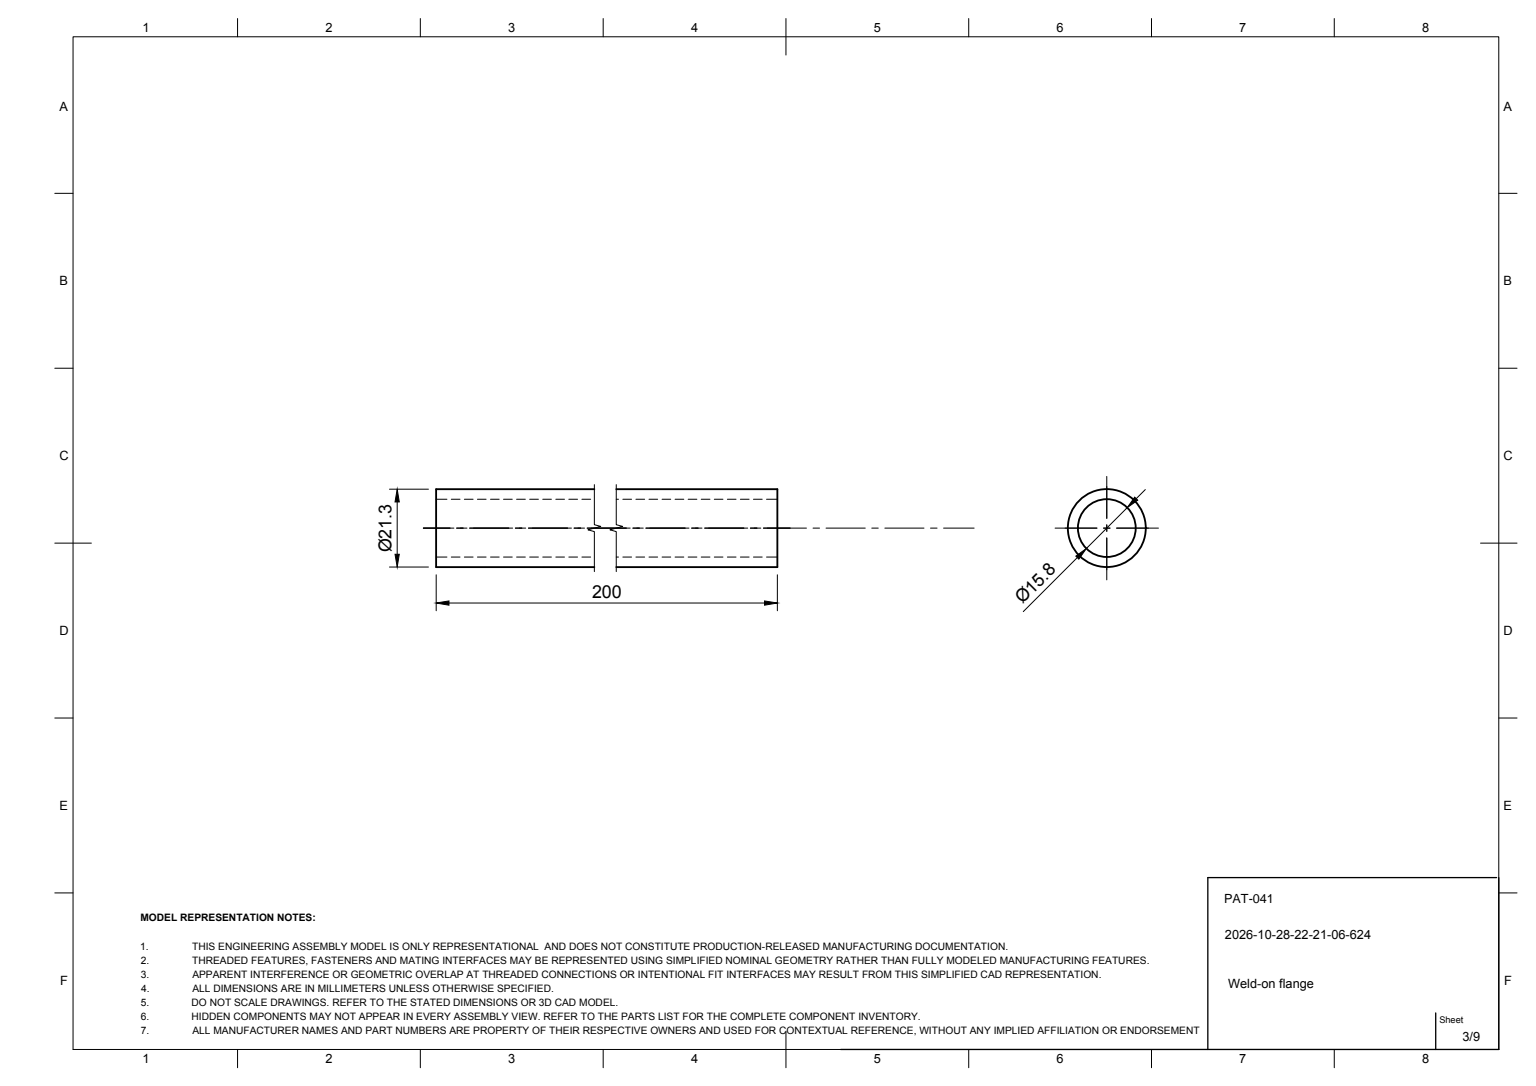
ISO-10303-21;
HEADER;
/* Generated by software containing ST-Developer
 * from STEP Tools, Inc. (www.steptools.com) 
 */

FILE_DESCRIPTION(
/* description */ ('PAT-041'),
/* implementation_level */ '2;1');

FILE_NAME(
/* name */ 'Weld-on flange.step',
/* time_stamp */ '2026-10-28T22:21:24-07:00',
/* author */ (''),
/* organization */ (''),
/* preprocessor_version */ 'ST-DEVELOPER v20.2',
/* originating_system */ 'Autodesk Translation Framework v15.17.0.0',
/* authorisation */ '');

FILE_SCHEMA (('AUTOMOTIVE_DESIGN { 1 0 10303 214 3 1 1 }'));
ENDSEC;

DATA;
#10=MECHANICAL_DESIGN_GEOMETRIC_PRESENTATION_REPRESENTATION('',(#210),#2507);
#190=SHAPE_REPRESENTATION_RELATIONSHIP('SRR','None',#2575,#200);
#200=ADVANCED_BREP_SHAPE_REPRESENTATION('',(#220),#2498);
#210=STYLED_ITEM('',(#2687),#220);
#220=MANIFOLD_SOLID_BREP('Body1',#1330);
#231=FACE_BOUND('',#397,.T.);
#232=FACE_BOUND('',#398,.T.);
#233=FACE_BOUND('',#399,.T.);
#234=FACE_BOUND('',#400,.T.);
#235=FACE_BOUND('',#401,.T.);
#236=FACE_BOUND('',#403,.T.);
#237=FACE_BOUND('',#404,.T.);
#238=FACE_BOUND('',#405,.T.);
#239=FACE_BOUND('',#406,.T.);
#240=FACE_BOUND('',#407,.T.);
#282=PLANE('',#1479);
#283=PLANE('',#1480);
#317=FACE_OUTER_BOUND('',#390,.T.);
#318=FACE_OUTER_BOUND('',#391,.T.);
#319=FACE_OUTER_BOUND('',#392,.T.);
#320=FACE_OUTER_BOUND('',#393,.T.);
#321=FACE_OUTER_BOUND('',#394,.T.);
#322=FACE_OUTER_BOUND('',#395,.T.);
#323=FACE_OUTER_BOUND('',#396,.T.);
#324=FACE_OUTER_BOUND('',#402,.T.);
#390=EDGE_LOOP('',(#944,#945,#946,#947));
#391=EDGE_LOOP('',(#948,#949,#950,#951));
#392=EDGE_LOOP('',(#952,#953,#954,#955));
#393=EDGE_LOOP('',(#956,#957,#958,#959));
#394=EDGE_LOOP('',(#960,#961,#962,#963));
#395=EDGE_LOOP('',(#964,#965,#966,#967));
#396=EDGE_LOOP('',(#968));
#397=EDGE_LOOP('',(#969));
#398=EDGE_LOOP('',(#970));
#399=EDGE_LOOP('',(#971));
#400=EDGE_LOOP('',(#972));
#401=EDGE_LOOP('',(#973));
#402=EDGE_LOOP('',(#974));
#403=EDGE_LOOP('',(#975));
#404=EDGE_LOOP('',(#976));
#405=EDGE_LOOP('',(#977));
#406=EDGE_LOOP('',(#978));
#407=EDGE_LOOP('',(#979));
#508=LINE('',#2106,#564);
#509=LINE('',#2112,#565);
#510=LINE('',#2118,#566);
#511=LINE('',#2124,#567);
#512=LINE('',#2130,#568);
#513=LINE('',#2136,#569);
#564=VECTOR('',#1671,0.44);
#565=VECTOR('',#1678,0.44);
#566=VECTOR('',#1685,0.44);
#567=VECTOR('',#1692,0.44);
#568=VECTOR('',#1699,1.065);
#569=VECTOR('',#1706,3.5);
#622=CIRCLE('',#1462,0.44);
#623=CIRCLE('',#1463,0.44);
#624=CIRCLE('',#1465,0.44);
#625=CIRCLE('',#1466,0.44);
#626=CIRCLE('',#1468,0.44);
#627=CIRCLE('',#1469,0.44);
#628=CIRCLE('',#1471,0.44);
#629=CIRCLE('',#1472,0.44);
#630=CIRCLE('',#1474,1.065);
#631=CIRCLE('',#1475,1.065);
#632=CIRCLE('',#1477,3.5);
#633=CIRCLE('',#1478,3.5);
#694=VERTEX_POINT('',#2103);
#695=VERTEX_POINT('',#2105);
#696=VERTEX_POINT('',#2109);
#697=VERTEX_POINT('',#2111);
#698=VERTEX_POINT('',#2115);
#699=VERTEX_POINT('',#2117);
#700=VERTEX_POINT('',#2121);
#701=VERTEX_POINT('',#2123);
#702=VERTEX_POINT('',#2127);
#703=VERTEX_POINT('',#2129);
#704=VERTEX_POINT('',#2133);
#705=VERTEX_POINT('',#2135);
#792=EDGE_CURVE('',#694,#694,#622,.T.);
#793=EDGE_CURVE('',#694,#695,#508,.T.);
#794=EDGE_CURVE('',#695,#695,#623,.T.);
#795=EDGE_CURVE('',#696,#696,#624,.T.);
#796=EDGE_CURVE('',#696,#697,#509,.T.);
#797=EDGE_CURVE('',#697,#697,#625,.T.);
#798=EDGE_CURVE('',#698,#698,#626,.T.);
#799=EDGE_CURVE('',#698,#699,#510,.T.);
#800=EDGE_CURVE('',#699,#699,#627,.T.);
#801=EDGE_CURVE('',#700,#700,#628,.T.);
#802=EDGE_CURVE('',#700,#701,#511,.T.);
#803=EDGE_CURVE('',#701,#701,#629,.T.);
#804=EDGE_CURVE('',#702,#702,#630,.T.);
#805=EDGE_CURVE('',#702,#703,#512,.T.);
#806=EDGE_CURVE('',#703,#703,#631,.T.);
#807=EDGE_CURVE('',#704,#704,#632,.T.);
#808=EDGE_CURVE('',#704,#705,#513,.T.);
#809=EDGE_CURVE('',#705,#705,#633,.T.);
#944=ORIENTED_EDGE('',*,*,#792,.F.);
#945=ORIENTED_EDGE('',*,*,#793,.T.);
#946=ORIENTED_EDGE('',*,*,#794,.F.);
#947=ORIENTED_EDGE('',*,*,#793,.F.);
#948=ORIENTED_EDGE('',*,*,#795,.F.);
#949=ORIENTED_EDGE('',*,*,#796,.T.);
#950=ORIENTED_EDGE('',*,*,#797,.F.);
#951=ORIENTED_EDGE('',*,*,#796,.F.);
#952=ORIENTED_EDGE('',*,*,#798,.F.);
#953=ORIENTED_EDGE('',*,*,#799,.T.);
#954=ORIENTED_EDGE('',*,*,#800,.F.);
#955=ORIENTED_EDGE('',*,*,#799,.F.);
#956=ORIENTED_EDGE('',*,*,#801,.F.);
#957=ORIENTED_EDGE('',*,*,#802,.T.);
#958=ORIENTED_EDGE('',*,*,#803,.F.);
#959=ORIENTED_EDGE('',*,*,#802,.F.);
#960=ORIENTED_EDGE('',*,*,#804,.F.);
#961=ORIENTED_EDGE('',*,*,#805,.T.);
#962=ORIENTED_EDGE('',*,*,#806,.T.);
#963=ORIENTED_EDGE('',*,*,#805,.F.);
#964=ORIENTED_EDGE('',*,*,#807,.F.);
#965=ORIENTED_EDGE('',*,*,#808,.T.);
#966=ORIENTED_EDGE('',*,*,#809,.T.);
#967=ORIENTED_EDGE('',*,*,#808,.F.);
#968=ORIENTED_EDGE('',*,*,#807,.T.);
#969=ORIENTED_EDGE('',*,*,#804,.T.);
#970=ORIENTED_EDGE('',*,*,#803,.T.);
#971=ORIENTED_EDGE('',*,*,#800,.T.);
#972=ORIENTED_EDGE('',*,*,#797,.T.);
#973=ORIENTED_EDGE('',*,*,#794,.T.);
#974=ORIENTED_EDGE('',*,*,#809,.F.);
#975=ORIENTED_EDGE('',*,*,#806,.F.);
#976=ORIENTED_EDGE('',*,*,#801,.T.);
#977=ORIENTED_EDGE('',*,*,#798,.T.);
#978=ORIENTED_EDGE('',*,*,#795,.T.);
#979=ORIENTED_EDGE('',*,*,#792,.T.);
#1226=CYLINDRICAL_SURFACE('',#1461,0.44);
#1227=CYLINDRICAL_SURFACE('',#1464,0.44);
#1228=CYLINDRICAL_SURFACE('',#1467,0.44);
#1229=CYLINDRICAL_SURFACE('',#1470,0.44);
#1230=CYLINDRICAL_SURFACE('',#1473,1.065);
#1231=CYLINDRICAL_SURFACE('',#1476,3.5);
#1262=ADVANCED_FACE('',(#317),#1226,.F.);
#1263=ADVANCED_FACE('',(#318),#1227,.F.);
#1264=ADVANCED_FACE('',(#319),#1228,.F.);
#1265=ADVANCED_FACE('',(#320),#1229,.F.);
#1266=ADVANCED_FACE('',(#321),#1230,.F.);
#1267=ADVANCED_FACE('',(#322),#1231,.T.);
#1268=ADVANCED_FACE('',(#323,#231,#232,#233,#234,#235),#282,.T.);
#1269=ADVANCED_FACE('',(#324,#236,#237,#238,#239,#240),#283,.F.);
#1330=CLOSED_SHELL('',(#1262,#1263,#1264,#1265,#1266,#1267,#1268,#1269));
#1460=AXIS2_PLACEMENT_3D('',#2101,#1665,#1666);
#1461=AXIS2_PLACEMENT_3D('',#2102,#1667,#1668);
#1462=AXIS2_PLACEMENT_3D('',#2104,#1669,#1670);
#1463=AXIS2_PLACEMENT_3D('',#2107,#1672,#1673);
#1464=AXIS2_PLACEMENT_3D('',#2108,#1674,#1675);
#1465=AXIS2_PLACEMENT_3D('',#2110,#1676,#1677);
#1466=AXIS2_PLACEMENT_3D('',#2113,#1679,#1680);
#1467=AXIS2_PLACEMENT_3D('',#2114,#1681,#1682);
#1468=AXIS2_PLACEMENT_3D('',#2116,#1683,#1684);
#1469=AXIS2_PLACEMENT_3D('',#2119,#1686,#1687);
#1470=AXIS2_PLACEMENT_3D('',#2120,#1688,#1689);
#1471=AXIS2_PLACEMENT_3D('',#2122,#1690,#1691);
#1472=AXIS2_PLACEMENT_3D('',#2125,#1693,#1694);
#1473=AXIS2_PLACEMENT_3D('',#2126,#1695,#1696);
#1474=AXIS2_PLACEMENT_3D('',#2128,#1697,#1698);
#1475=AXIS2_PLACEMENT_3D('',#2131,#1700,#1701);
#1476=AXIS2_PLACEMENT_3D('',#2132,#1702,#1703);
#1477=AXIS2_PLACEMENT_3D('',#2134,#1704,#1705);
#1478=AXIS2_PLACEMENT_3D('',#2137,#1707,#1708);
#1479=AXIS2_PLACEMENT_3D('',#2138,#1709,#1710);
#1480=AXIS2_PLACEMENT_3D('',#2139,#1711,#1712);
#1665=DIRECTION('axis',(0.,0.,1.));
#1666=DIRECTION('refdir',(1.,0.,0.));
#1667=DIRECTION('center_axis',(1.,0.,0.));
#1668=DIRECTION('ref_axis',(0.,0.,-1.));
#1669=DIRECTION('center_axis',(1.,0.,0.));
#1670=DIRECTION('ref_axis',(0.,0.,-1.));
#1671=DIRECTION('',(1.,0.,0.));
#1672=DIRECTION('center_axis',(-1.,0.,0.));
#1673=DIRECTION('ref_axis',(0.,0.,-1.));
#1674=DIRECTION('center_axis',(1.,0.,0.));
#1675=DIRECTION('ref_axis',(0.,0.,-1.));
#1676=DIRECTION('center_axis',(1.,0.,0.));
#1677=DIRECTION('ref_axis',(0.,0.,-1.));
#1678=DIRECTION('',(1.,0.,0.));
#1679=DIRECTION('center_axis',(-1.,0.,0.));
#1680=DIRECTION('ref_axis',(0.,0.,-1.));
#1681=DIRECTION('center_axis',(1.,0.,0.));
#1682=DIRECTION('ref_axis',(0.,0.,-1.));
#1683=DIRECTION('center_axis',(1.,0.,0.));
#1684=DIRECTION('ref_axis',(0.,0.,-1.));
#1685=DIRECTION('',(1.,0.,0.));
#1686=DIRECTION('center_axis',(-1.,0.,0.));
#1687=DIRECTION('ref_axis',(0.,0.,-1.));
#1688=DIRECTION('center_axis',(1.,0.,0.));
#1689=DIRECTION('ref_axis',(0.,0.,-1.));
#1690=DIRECTION('center_axis',(1.,0.,0.));
#1691=DIRECTION('ref_axis',(0.,0.,-1.));
#1692=DIRECTION('',(1.,0.,0.));
#1693=DIRECTION('center_axis',(-1.,0.,0.));
#1694=DIRECTION('ref_axis',(0.,0.,-1.));
#1695=DIRECTION('center_axis',(1.,0.,0.));
#1696=DIRECTION('ref_axis',(0.,0.,-1.));
#1697=DIRECTION('center_axis',(-1.,0.,0.));
#1698=DIRECTION('ref_axis',(0.,0.,-1.));
#1699=DIRECTION('',(-1.,0.,0.));
#1700=DIRECTION('center_axis',(-1.,0.,0.));
#1701=DIRECTION('ref_axis',(0.,0.,-1.));
#1702=DIRECTION('center_axis',(1.,0.,0.));
#1703=DIRECTION('ref_axis',(0.,0.,-1.));
#1704=DIRECTION('center_axis',(1.,0.,0.));
#1705=DIRECTION('ref_axis',(0.,0.,-1.));
#1706=DIRECTION('',(-1.,0.,0.));
#1707=DIRECTION('center_axis',(1.,0.,0.));
#1708=DIRECTION('ref_axis',(0.,0.,-1.));
#1709=DIRECTION('center_axis',(1.,0.,0.));
#1710=DIRECTION('ref_axis',(0.,0.,-1.));
#1711=DIRECTION('center_axis',(1.,0.,0.));
#1712=DIRECTION('ref_axis',(0.,0.,-1.));
#2101=CARTESIAN_POINT('',(0.,0.,0.));
#2102=CARTESIAN_POINT('Origin',(-10.1,-1.90918830920368,-1.90918830920368));
#2103=CARTESIAN_POINT('',(-10.,-1.90918830920368,-1.46918830920368));
#2104=CARTESIAN_POINT('Origin',(-10.,-1.90918830920368,-1.90918830920368));
#2105=CARTESIAN_POINT('',(-9.2,-1.90918830920368,-1.46918830920368));
#2106=CARTESIAN_POINT('',(-10.1,-1.90918830920368,-1.46918830920368));
#2107=CARTESIAN_POINT('Origin',(-9.2,-1.90918830920368,-1.90918830920368));
#2108=CARTESIAN_POINT('Origin',(-10.1,-1.90918830920368,1.90918830920368));
#2109=CARTESIAN_POINT('',(-10.,-1.90918830920368,2.34918830920368));
#2110=CARTESIAN_POINT('Origin',(-10.,-1.90918830920368,1.90918830920368));
#2111=CARTESIAN_POINT('',(-9.2,-1.90918830920368,2.34918830920368));
#2112=CARTESIAN_POINT('',(-10.1,-1.90918830920368,2.34918830920368));
#2113=CARTESIAN_POINT('Origin',(-9.2,-1.90918830920368,1.90918830920368));
#2114=CARTESIAN_POINT('Origin',(-10.1,1.90918830920368,1.90918830920368));
#2115=CARTESIAN_POINT('',(-10.,1.90918830920368,2.34918830920368));
#2116=CARTESIAN_POINT('Origin',(-10.,1.90918830920368,1.90918830920368));
#2117=CARTESIAN_POINT('',(-9.2,1.90918830920368,2.34918830920368));
#2118=CARTESIAN_POINT('',(-10.1,1.90918830920368,2.34918830920368));
#2119=CARTESIAN_POINT('Origin',(-9.2,1.90918830920368,1.90918830920368));
#2120=CARTESIAN_POINT('Origin',(-10.1,1.90918830920368,-1.90918830920368));
#2121=CARTESIAN_POINT('',(-10.,1.90918830920368,-1.46918830920368));
#2122=CARTESIAN_POINT('Origin',(-10.,1.90918830920368,-1.90918830920368));
#2123=CARTESIAN_POINT('',(-9.2,1.90918830920368,-1.46918830920368));
#2124=CARTESIAN_POINT('',(-10.1,1.90918830920368,-1.46918830920368));
#2125=CARTESIAN_POINT('Origin',(-9.2,1.90918830920368,-1.90918830920368));
#2126=CARTESIAN_POINT('Origin',(-10.,0.,0.));
#2127=CARTESIAN_POINT('',(-9.2,-1.30424884109193E-16,1.065));
#2128=CARTESIAN_POINT('Origin',(-9.2,0.,0.));
#2129=CARTESIAN_POINT('',(-10.,-1.30424884109193E-16,1.065));
#2130=CARTESIAN_POINT('',(-10.,-1.30424884109193E-16,1.065));
#2131=CARTESIAN_POINT('Origin',(-10.,0.,0.));
#2132=CARTESIAN_POINT('Origin',(-10.,0.,0.));
#2133=CARTESIAN_POINT('',(-9.2,-4.28626379701574E-16,3.5));
#2134=CARTESIAN_POINT('Origin',(-9.2,0.,0.));
#2135=CARTESIAN_POINT('',(-10.,-4.28626379701574E-16,3.5));
#2136=CARTESIAN_POINT('',(-10.,-4.28626379701574E-16,3.5));
#2137=CARTESIAN_POINT('Origin',(-10.,0.,0.));
#2138=CARTESIAN_POINT('Origin',(-9.2,0.,0.));
#2139=CARTESIAN_POINT('Origin',(-10.,0.,0.));
#2486=UNCERTAINTY_MEASURE_WITH_UNIT(LENGTH_MEASURE(0.001),#2508,
'DISTANCE_ACCURACY_VALUE',
'Maximum model space distance between geometric entities at asserted c
onnectivities');
#2495=UNCERTAINTY_MEASURE_WITH_UNIT(LENGTH_MEASURE(0.001),#2508,
'DISTANCE_ACCURACY_VALUE',
'Maximum model space distance between geometric entities at asserted c
onnectivities');
#2498=(
GEOMETRIC_REPRESENTATION_CONTEXT(3)
GLOBAL_UNCERTAINTY_ASSIGNED_CONTEXT((#2486))
GLOBAL_UNIT_ASSIGNED_CONTEXT((#2508,#2510,#2511))
REPRESENTATION_CONTEXT('','3D')
);
#2507=(
GEOMETRIC_REPRESENTATION_CONTEXT(3)
GLOBAL_UNCERTAINTY_ASSIGNED_CONTEXT((#2495))
GLOBAL_UNIT_ASSIGNED_CONTEXT((#2508,#2510,#2511))
REPRESENTATION_CONTEXT('','3D')
);
#2508=(
LENGTH_UNIT()
NAMED_UNIT(*)
SI_UNIT(.CENTI.,.METRE.)
);
#2510=(
NAMED_UNIT(*)
PLANE_ANGLE_UNIT()
SI_UNIT($,.RADIAN.)
);
#2511=(
NAMED_UNIT(*)
SI_UNIT($,.STERADIAN.)
SOLID_ANGLE_UNIT()
);
#2514=SHAPE_DEFINITION_REPRESENTATION(#2525,#2575);
#2525=PRODUCT_DEFINITION_SHAPE('',$,#2587);
#2575=SHAPE_REPRESENTATION('',(#1460),#2498);
#2584=PRODUCT_DEFINITION_CONTEXT('part definition',#2619,'design');
#2587=PRODUCT_DEFINITION('Weld-on flange','Weld-on flange',#2598,
#2584);
#2598=PRODUCT_DEFINITION_FORMATION('',$,#2623);
#2619=APPLICATION_CONTEXT(
'Core Data for Automotive Mechanical Design Process');
#2620=PRODUCT_CONTEXT('part definition',#2619,'mechanical');
#2623=PRODUCT('Weld-on flange','Weld-on flange',
'Weld-on flange',(#2620));
#2681=COLOUR_RGB('Sky Blue',0.24,0.69,0.87);
#2682=FILL_AREA_STYLE_COLOUR('',#2681);
#2683=FILL_AREA_STYLE('',(#2682));
#2684=SURFACE_STYLE_FILL_AREA(#2683);
#2685=SURFACE_SIDE_STYLE('',(#2684));
#2686=SURFACE_STYLE_USAGE(.BOTH.,#2685);
#2687=PRESENTATION_STYLE_ASSIGNMENT((#2686));
ENDSEC;
END-ISO-10303-21;
